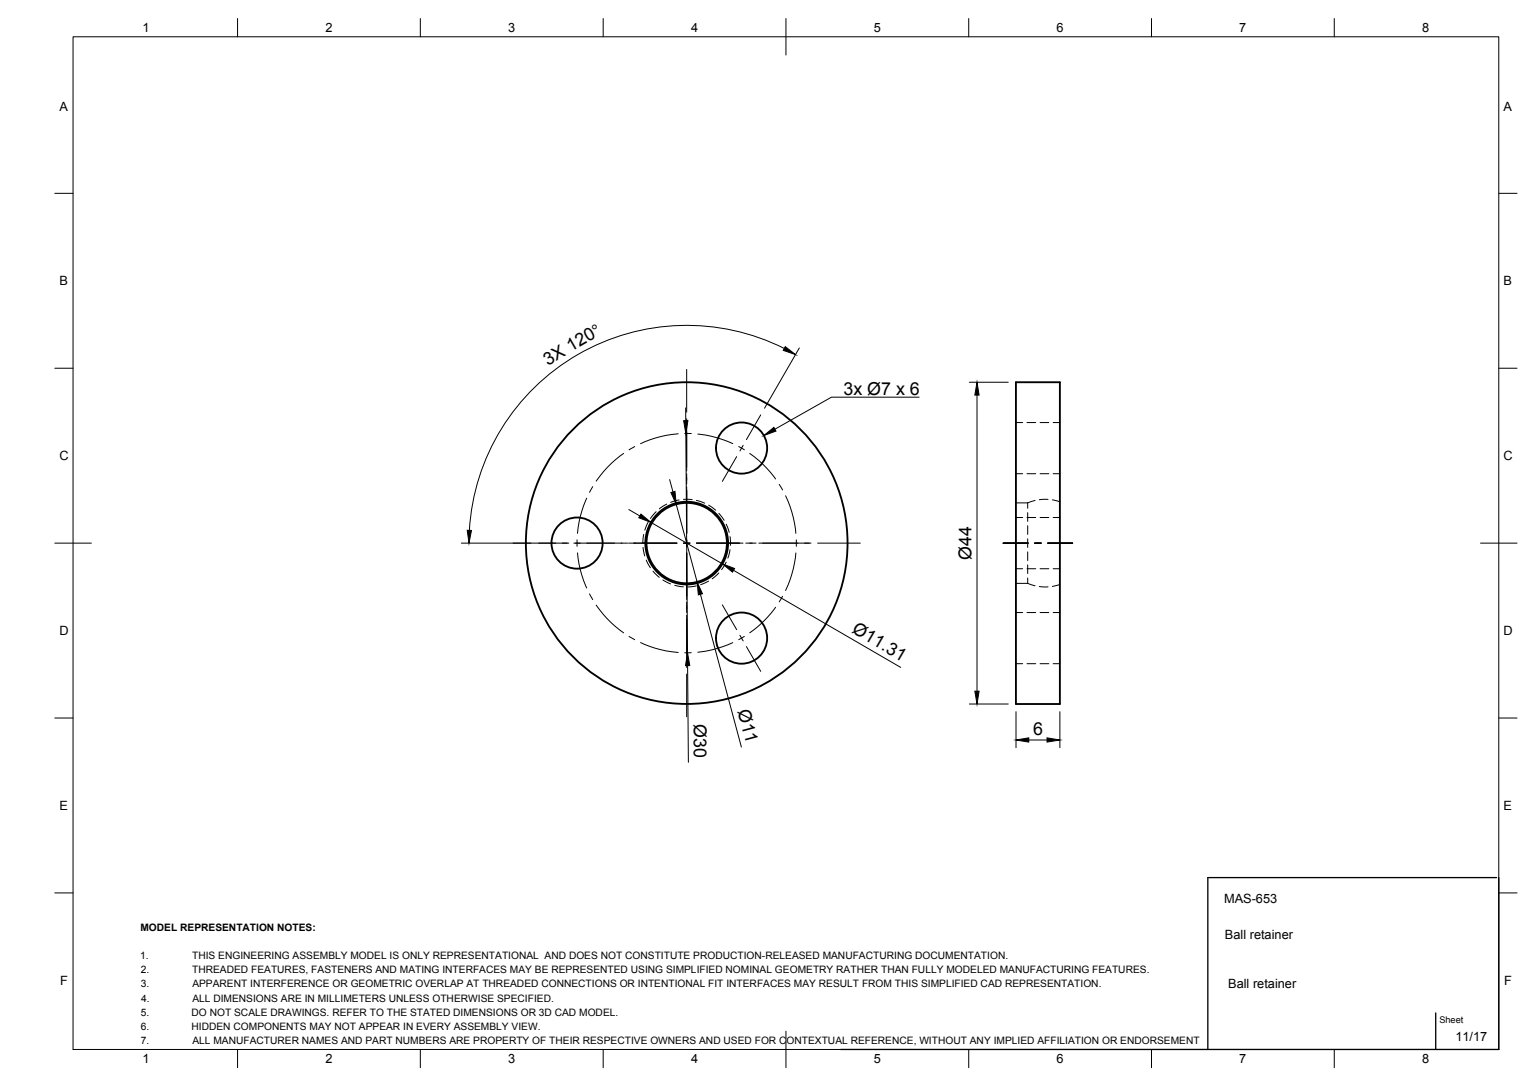
ISO-10303-21;
HEADER;
/* Generated by software containing ST-Developer
 * from STEP Tools, Inc. (www.steptools.com) 
 */

FILE_DESCRIPTION(
/* description */ ('Independent compact industrial fixture table, bolted aluminum worktop
 on connected adjustable support base. Whole-mm nominal dimensions. No
 load rating assigned.'),
/* implementation_level */ '2;1');

FILE_NAME(
/* name */ 'Ball retainer.step',
/* time_stamp */ '2026-11-07T17:47:58-08:00',
/* author */ (''),
/* organization */ (''),
/* preprocessor_version */ 'ST-DEVELOPER v20.2',
/* originating_system */ 'Autodesk Translation Framework v15.17.0.0',
/* authorisation */ '');

FILE_SCHEMA (('AUTOMOTIVE_DESIGN { 1 0 10303 214 3 1 1 }'));
ENDSEC;

DATA;
#10=MECHANICAL_DESIGN_GEOMETRIC_PRESENTATION_REPRESENTATION('',(#2260),#97475);
#12=SPHERICAL_SURFACE('',#22798,6.);
#2222=SHAPE_REPRESENTATION_RELATIONSHIP('SRR','None',#97616,#2241);
#2241=ADVANCED_BREP_SHAPE_REPRESENTATION('',(#2279),#97466);
#2260=STYLED_ITEM('',(#97719),#2279);
#2279=MANIFOLD_SOLID_BREP('Body1',#21821);
#2345=FACE_BOUND('',#4296,.T.);
#2346=FACE_BOUND('',#4297,.T.);
#2347=FACE_BOUND('',#4298,.T.);
#2348=FACE_BOUND('',#4299,.T.);
#2349=FACE_BOUND('',#4301,.T.);
#2350=FACE_BOUND('',#4302,.T.);
#2351=FACE_BOUND('',#4303,.T.);
#2352=FACE_BOUND('',#4304,.T.);
#2486=PLANE('',#22807);
#2487=PLANE('',#22808);
#3078=FACE_OUTER_BOUND('',#4289,.T.);
#3079=FACE_OUTER_BOUND('',#4290,.T.);
#3080=FACE_OUTER_BOUND('',#4291,.T.);
#3081=FACE_OUTER_BOUND('',#4292,.T.);
#3082=FACE_OUTER_BOUND('',#4293,.T.);
#3083=FACE_OUTER_BOUND('',#4294,.T.);
#3084=FACE_OUTER_BOUND('',#4295,.T.);
#3085=FACE_OUTER_BOUND('',#4300,.T.);
#4289=EDGE_LOOP('',(#16176,#16177,#16178,#16179));
#4290=EDGE_LOOP('',(#16180,#16181,#16182,#16183));
#4291=EDGE_LOOP('',(#16184,#16185,#16186,#16187));
#4292=EDGE_LOOP('',(#16188,#16189,#16190,#16191));
#4293=EDGE_LOOP('',(#16192,#16193,#16194,#16195));
#4294=EDGE_LOOP('',(#16196,#16197,#16198,#16199));
#4295=EDGE_LOOP('',(#16200));
#4296=EDGE_LOOP('',(#16201));
#4297=EDGE_LOOP('',(#16202));
#4298=EDGE_LOOP('',(#16203));
#4299=EDGE_LOOP('',(#16204));
#4300=EDGE_LOOP('',(#16205));
#4301=EDGE_LOOP('',(#16206));
#4302=EDGE_LOOP('',(#16207));
#4303=EDGE_LOOP('',(#16208));
#4304=EDGE_LOOP('',(#16209));
#5546=LINE('',#60812,#6760);
#5547=LINE('',#60818,#6761);
#5548=LINE('',#60824,#6762);
#5549=LINE('',#60835,#6763);
#5550=LINE('',#60840,#6764);
#6760=VECTOR('',#25614,3.5);
#6761=VECTOR('',#25621,3.5);
#6762=VECTOR('',#25628,3.5);
#6763=VECTOR('',#25643,5.5);
#6764=VECTOR('',#25648,22.);
#7540=CIRCLE('',#22790,3.5);
#7541=CIRCLE('',#22791,3.5);
#7542=CIRCLE('',#22793,3.5);
#7543=CIRCLE('',#22794,3.5);
#7544=CIRCLE('',#22796,3.5);
#7545=CIRCLE('',#22797,3.5);
#7546=CIRCLE('',#22799,5.65685424949238);
#7547=CIRCLE('',#22800,6.);
#7548=CIRCLE('',#22801,5.5);
#7549=CIRCLE('',#22803,5.5);
#7550=CIRCLE('',#22805,22.);
#7551=CIRCLE('',#22806,22.);
#8635=VERTEX_POINT('',#60809);
#8636=VERTEX_POINT('',#60811);
#8637=VERTEX_POINT('',#60815);
#8638=VERTEX_POINT('',#60817);
#8639=VERTEX_POINT('',#60821);
#8640=VERTEX_POINT('',#60823);
#8641=VERTEX_POINT('',#60827);
#8642=VERTEX_POINT('',#60829);
#8643=VERTEX_POINT('',#60833);
#8644=VERTEX_POINT('',#60837);
#8645=VERTEX_POINT('',#60839);
#11345=EDGE_CURVE('',#8635,#8635,#7540,.T.);
#11346=EDGE_CURVE('',#8635,#8636,#5546,.T.);
#11347=EDGE_CURVE('',#8636,#8636,#7541,.T.);
#11348=EDGE_CURVE('',#8637,#8637,#7542,.T.);
#11349=EDGE_CURVE('',#8637,#8638,#5547,.T.);
#11350=EDGE_CURVE('',#8638,#8638,#7543,.T.);
#11351=EDGE_CURVE('',#8639,#8639,#7544,.T.);
#11352=EDGE_CURVE('',#8639,#8640,#5548,.T.);
#11353=EDGE_CURVE('',#8640,#8640,#7545,.T.);
#11354=EDGE_CURVE('',#8641,#8641,#7546,.T.);
#11355=EDGE_CURVE('',#8641,#8642,#7547,.T.);
#11356=EDGE_CURVE('',#8642,#8642,#7548,.T.);
#11357=EDGE_CURVE('',#8643,#8643,#7549,.T.);
#11358=EDGE_CURVE('',#8643,#8642,#5549,.T.);
#11359=EDGE_CURVE('',#8644,#8644,#7550,.T.);
#11360=EDGE_CURVE('',#8644,#8645,#5550,.T.);
#11361=EDGE_CURVE('',#8645,#8645,#7551,.T.);
#16176=ORIENTED_EDGE('',*,*,#11345,.F.);
#16177=ORIENTED_EDGE('',*,*,#11346,.T.);
#16178=ORIENTED_EDGE('',*,*,#11347,.F.);
#16179=ORIENTED_EDGE('',*,*,#11346,.F.);
#16180=ORIENTED_EDGE('',*,*,#11348,.F.);
#16181=ORIENTED_EDGE('',*,*,#11349,.T.);
#16182=ORIENTED_EDGE('',*,*,#11350,.F.);
#16183=ORIENTED_EDGE('',*,*,#11349,.F.);
#16184=ORIENTED_EDGE('',*,*,#11351,.F.);
#16185=ORIENTED_EDGE('',*,*,#11352,.T.);
#16186=ORIENTED_EDGE('',*,*,#11353,.F.);
#16187=ORIENTED_EDGE('',*,*,#11352,.F.);
#16188=ORIENTED_EDGE('',*,*,#11354,.F.);
#16189=ORIENTED_EDGE('',*,*,#11355,.T.);
#16190=ORIENTED_EDGE('',*,*,#11356,.F.);
#16191=ORIENTED_EDGE('',*,*,#11355,.F.);
#16192=ORIENTED_EDGE('',*,*,#11357,.F.);
#16193=ORIENTED_EDGE('',*,*,#11358,.T.);
#16194=ORIENTED_EDGE('',*,*,#11356,.T.);
#16195=ORIENTED_EDGE('',*,*,#11358,.F.);
#16196=ORIENTED_EDGE('',*,*,#11359,.F.);
#16197=ORIENTED_EDGE('',*,*,#11360,.T.);
#16198=ORIENTED_EDGE('',*,*,#11361,.T.);
#16199=ORIENTED_EDGE('',*,*,#11360,.F.);
#16200=ORIENTED_EDGE('',*,*,#11359,.T.);
#16201=ORIENTED_EDGE('',*,*,#11345,.T.);
#16202=ORIENTED_EDGE('',*,*,#11348,.T.);
#16203=ORIENTED_EDGE('',*,*,#11351,.T.);
#16204=ORIENTED_EDGE('',*,*,#11357,.T.);
#16205=ORIENTED_EDGE('',*,*,#11361,.F.);
#16206=ORIENTED_EDGE('',*,*,#11347,.T.);
#16207=ORIENTED_EDGE('',*,*,#11350,.T.);
#16208=ORIENTED_EDGE('',*,*,#11353,.T.);
#16209=ORIENTED_EDGE('',*,*,#11354,.T.);
#20119=CYLINDRICAL_SURFACE('',#22789,3.5);
#20120=CYLINDRICAL_SURFACE('',#22792,3.5);
#20121=CYLINDRICAL_SURFACE('',#22795,3.5);
#20122=CYLINDRICAL_SURFACE('',#22802,5.5);
#20123=CYLINDRICAL_SURFACE('',#22804,22.);
#21198=ADVANCED_FACE('',(#3078),#20119,.F.);
#21199=ADVANCED_FACE('',(#3079),#20120,.F.);
#21200=ADVANCED_FACE('',(#3080),#20121,.F.);
#21201=ADVANCED_FACE('',(#3081),#12,.F.);
#21202=ADVANCED_FACE('',(#3082),#20122,.F.);
#21203=ADVANCED_FACE('',(#3083),#20123,.T.);
#21204=ADVANCED_FACE('',(#3084,#2345,#2346,#2347,#2348),#2486,.T.);
#21205=ADVANCED_FACE('',(#3085,#2349,#2350,#2351,#2352),#2487,.F.);
#21821=CLOSED_SHELL('',(#21198,#21199,#21200,#21201,#21202,#21203,#21204,
#21205));
#22788=AXIS2_PLACEMENT_3D('',#60807,#25608,#25609);
#22789=AXIS2_PLACEMENT_3D('',#60808,#25610,#25611);
#22790=AXIS2_PLACEMENT_3D('',#60810,#25612,#25613);
#22791=AXIS2_PLACEMENT_3D('',#60813,#25615,#25616);
#22792=AXIS2_PLACEMENT_3D('',#60814,#25617,#25618);
#22793=AXIS2_PLACEMENT_3D('',#60816,#25619,#25620);
#22794=AXIS2_PLACEMENT_3D('',#60819,#25622,#25623);
#22795=AXIS2_PLACEMENT_3D('',#60820,#25624,#25625);
#22796=AXIS2_PLACEMENT_3D('',#60822,#25626,#25627);
#22797=AXIS2_PLACEMENT_3D('',#60825,#25629,#25630);
#22798=AXIS2_PLACEMENT_3D('',#60826,#25631,#25632);
#22799=AXIS2_PLACEMENT_3D('',#60828,#25633,#25634);
#22800=AXIS2_PLACEMENT_3D('',#60830,#25635,#25636);
#22801=AXIS2_PLACEMENT_3D('',#60831,#25637,#25638);
#22802=AXIS2_PLACEMENT_3D('',#60832,#25639,#25640);
#22803=AXIS2_PLACEMENT_3D('',#60834,#25641,#25642);
#22804=AXIS2_PLACEMENT_3D('',#60836,#25644,#25645);
#22805=AXIS2_PLACEMENT_3D('',#60838,#25646,#25647);
#22806=AXIS2_PLACEMENT_3D('',#60841,#25649,#25650);
#22807=AXIS2_PLACEMENT_3D('',#60842,#25651,#25652);
#22808=AXIS2_PLACEMENT_3D('',#60843,#25653,#25654);
#25608=DIRECTION('axis',(0.,0.,1.));
#25609=DIRECTION('refdir',(1.,0.,0.));
#25610=DIRECTION('center_axis',(0.,0.,-1.));
#25611=DIRECTION('ref_axis',(1.,0.,0.));
#25612=DIRECTION('center_axis',(0.,0.,-1.));
#25613=DIRECTION('ref_axis',(1.,0.,0.));
#25614=DIRECTION('',(0.,0.,-1.));
#25615=DIRECTION('center_axis',(0.,0.,1.));
#25616=DIRECTION('ref_axis',(1.,0.,0.));
#25617=DIRECTION('center_axis',(0.,0.,-1.));
#25618=DIRECTION('ref_axis',(1.,0.,0.));
#25619=DIRECTION('center_axis',(0.,0.,-1.));
#25620=DIRECTION('ref_axis',(1.,0.,0.));
#25621=DIRECTION('',(0.,0.,-1.));
#25622=DIRECTION('center_axis',(0.,0.,1.));
#25623=DIRECTION('ref_axis',(1.,0.,0.));
#25624=DIRECTION('center_axis',(0.,0.,-1.));
#25625=DIRECTION('ref_axis',(1.,0.,0.));
#25626=DIRECTION('center_axis',(0.,0.,-1.));
#25627=DIRECTION('ref_axis',(1.,0.,0.));
#25628=DIRECTION('',(0.,0.,-1.));
#25629=DIRECTION('center_axis',(0.,0.,1.));
#25630=DIRECTION('ref_axis',(1.,0.,0.));
#25631=DIRECTION('center_axis',(6.12323399573677E-17,0.,1.));
#25632=DIRECTION('ref_axis',(1.,0.,0.));
#25633=DIRECTION('center_axis',(0.,0.,1.));
#25634=DIRECTION('ref_axis',(0.,-1.,0.));
#25635=DIRECTION('center_axis',(-1.22464679914735E-16,1.,0.));
#25636=DIRECTION('ref_axis',(-1.,-1.22464679914735E-16,0.));
#25637=DIRECTION('center_axis',(0.,0.,-1.));
#25638=DIRECTION('ref_axis',(1.,0.,0.));
#25639=DIRECTION('center_axis',(0.,0.,1.));
#25640=DIRECTION('ref_axis',(1.,0.,0.));
#25641=DIRECTION('center_axis',(0.,0.,-1.));
#25642=DIRECTION('ref_axis',(1.,0.,0.));
#25643=DIRECTION('',(0.,0.,-1.));
#25644=DIRECTION('center_axis',(0.,0.,1.));
#25645=DIRECTION('ref_axis',(1.,0.,0.));
#25646=DIRECTION('center_axis',(0.,0.,1.));
#25647=DIRECTION('ref_axis',(1.,0.,0.));
#25648=DIRECTION('',(0.,0.,-1.));
#25649=DIRECTION('center_axis',(0.,0.,1.));
#25650=DIRECTION('ref_axis',(1.,0.,0.));
#25651=DIRECTION('center_axis',(0.,0.,1.));
#25652=DIRECTION('ref_axis',(1.,0.,0.));
#25653=DIRECTION('center_axis',(0.,0.,1.));
#25654=DIRECTION('ref_axis',(1.,0.,0.));
#60807=CARTESIAN_POINT('',(0.,0.,0.));
#60808=CARTESIAN_POINT('Origin',(-7.5,12.9903810567666,15.));
#60809=CARTESIAN_POINT('',(-11.,12.9903810567666,18.));
#60810=CARTESIAN_POINT('Origin',(-7.5,12.9903810567666,18.));
#60811=CARTESIAN_POINT('',(-11.,12.9903810567666,12.));
#60812=CARTESIAN_POINT('',(-11.,12.9903810567666,15.));
#60813=CARTESIAN_POINT('Origin',(-7.5,12.9903810567666,12.));
#60814=CARTESIAN_POINT('Origin',(15.,0.,15.));
#60815=CARTESIAN_POINT('',(11.5,4.28626379701574E-16,18.));
#60816=CARTESIAN_POINT('Origin',(15.,0.,18.));
#60817=CARTESIAN_POINT('',(11.5,4.28626379701574E-16,12.));
#60818=CARTESIAN_POINT('',(11.5,4.28626379701574E-16,15.));
#60819=CARTESIAN_POINT('Origin',(15.,0.,12.));
#60820=CARTESIAN_POINT('Origin',(-7.50000000000001,-12.9903810567666,15.));
#60821=CARTESIAN_POINT('',(-11.,-12.9903810567666,18.));
#60822=CARTESIAN_POINT('Origin',(-7.50000000000001,-12.9903810567666,18.));
#60823=CARTESIAN_POINT('',(-11.,-12.9903810567666,12.));
#60824=CARTESIAN_POINT('',(-11.,-12.9903810567666,15.));
#60825=CARTESIAN_POINT('Origin',(-7.50000000000001,-12.9903810567666,12.));
#60826=CARTESIAN_POINT('Origin',(5.55111512312578E-16,0.,14.));
#60827=CARTESIAN_POINT('',(-5.65685424949238,-6.92764844988394E-16,12.));
#60828=CARTESIAN_POINT('Origin',(5.55111512312578E-16,0.,12.));
#60829=CARTESIAN_POINT('',(-5.5,6.73555739531044E-16,16.3979157616564));
#60830=CARTESIAN_POINT('Origin',(5.55111512312578E-16,0.,14.));
#60831=CARTESIAN_POINT('Origin',(0.,0.,16.3979157616564));
#60832=CARTESIAN_POINT('Origin',(0.,0.,12.));
#60833=CARTESIAN_POINT('',(-5.5,-6.73555739531044E-16,18.));
#60834=CARTESIAN_POINT('Origin',(0.,0.,18.));
#60835=CARTESIAN_POINT('',(-5.5,-6.73555739531044E-16,12.));
#60836=CARTESIAN_POINT('Origin',(0.,0.,12.));
#60837=CARTESIAN_POINT('',(-22.,-2.69422295812418E-15,18.));
#60838=CARTESIAN_POINT('Origin',(0.,0.,18.));
#60839=CARTESIAN_POINT('',(-22.,-2.69422295812418E-15,12.));
#60840=CARTESIAN_POINT('',(-22.,-2.69422295812418E-15,12.));
#60841=CARTESIAN_POINT('Origin',(0.,0.,12.));
#60842=CARTESIAN_POINT('Origin',(0.,0.,18.));
#60843=CARTESIAN_POINT('Origin',(0.,0.,12.));
#97443=UNCERTAINTY_MEASURE_WITH_UNIT(LENGTH_MEASURE(0.01),#97476,
'DISTANCE_ACCURACY_VALUE',
'Maximum model space distance between geometric entities at asserted c
onnectivities');
#97452=UNCERTAINTY_MEASURE_WITH_UNIT(LENGTH_MEASURE(0.01),#97476,
'DISTANCE_ACCURACY_VALUE',
'Maximum model space distance between geometric entities at asserted c
onnectivities');
#97466=(
GEOMETRIC_REPRESENTATION_CONTEXT(3)
GLOBAL_UNCERTAINTY_ASSIGNED_CONTEXT((#97443))
GLOBAL_UNIT_ASSIGNED_CONTEXT((#97476,#97478,#97479))
REPRESENTATION_CONTEXT('','3D')
);
#97475=(
GEOMETRIC_REPRESENTATION_CONTEXT(3)
GLOBAL_UNCERTAINTY_ASSIGNED_CONTEXT((#97452))
GLOBAL_UNIT_ASSIGNED_CONTEXT((#97476,#97478,#97479))
REPRESENTATION_CONTEXT('','3D')
);
#97476=(
LENGTH_UNIT()
NAMED_UNIT(*)
SI_UNIT(.MILLI.,.METRE.)
);
#97478=(
NAMED_UNIT(*)
PLANE_ANGLE_UNIT()
SI_UNIT($,.RADIAN.)
);
#97479=(
NAMED_UNIT(*)
SI_UNIT($,.STERADIAN.)
SOLID_ANGLE_UNIT()
);
#97493=SHAPE_DEFINITION_REPRESENTATION(#97555,#97616);
#97555=PRODUCT_DEFINITION_SHAPE('',$,#97639);
#97616=SHAPE_REPRESENTATION('',(#22788),#97466);
#97625=PRODUCT_DEFINITION_CONTEXT('part definition',#97693,'design');
#97639=PRODUCT_DEFINITION('Ball retainer','Ball retainer',#97661,#97625);
#97661=PRODUCT_DEFINITION_FORMATION('',$,#97708);
#97693=APPLICATION_CONTEXT(
'Core Data for Automotive Mechanical Design Process');
#97694=PRODUCT_CONTEXT('part definition',#97693,'mechanical');
#97708=PRODUCT('Ball retainer','Ball retainer',$,(#97694));
#97719=PRESENTATION_STYLE_ASSIGNMENT((#97726));
#97726=SURFACE_STYLE_USAGE(.BOTH.,#97733);
#97733=SURFACE_SIDE_STYLE('',(#97740));
#97740=SURFACE_STYLE_FILL_AREA(#97747);
#97747=FILL_AREA_STYLE('Sky blue',(#97754));
#97754=FILL_AREA_STYLE_COLOUR('Sky blue',#97761);
#97761=COLOUR_RGB('Sky blue',0.317647058823529,0.686274509803922,0.890196078431372);
ENDSEC;
END-ISO-10303-21;
